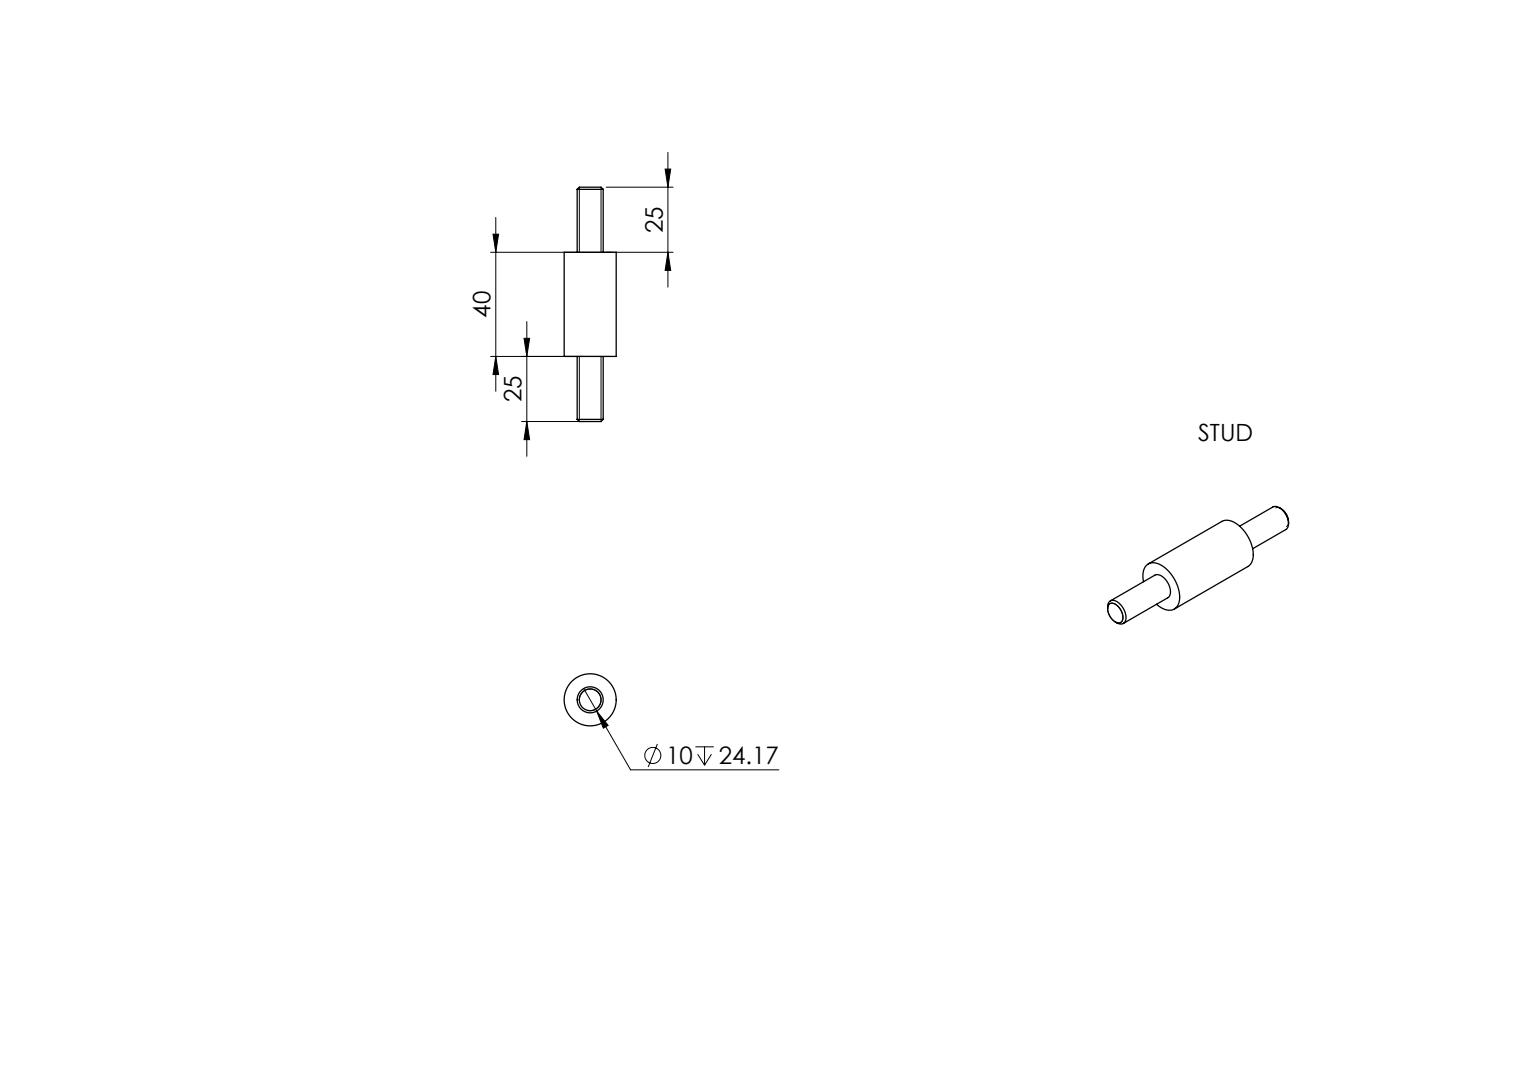
ISO-10303-21;
HEADER;
FILE_DESCRIPTION (('STEP AP214'),
    '1' );
FILE_NAME ('stud.step',
    '2026-10-23T05:12:30',
    ( '' ),
    ( '' ),
    'SwSTEP 2.0',
    'SolidWorks 2026',
    '' );
FILE_SCHEMA (( 'AUTOMOTIVE_DESIGN' ));
ENDSEC;

DATA;
#14=ORIENTED_EDGE ( 'NONE', *, *, #6597, .T. ) ;
#88=ADVANCED_FACE ( 'NONE', ( #7673 ), #6574, .T. ) ;
#119=CIRCLE ( 'NONE', #3022, 10.00000000000000178 ) ;
#120=DIRECTION ( 'NONE',  ( -0.000000000000000000, -0.000000000000000000, 1.000000000000000000 ) ) ;
#168=CIRCLE ( 'NONE', #5710, 4.171999999999995268 ) ;
#219=VERTEX_POINT ( 'NONE', #3065 ) ;
#231=VECTOR ( 'NONE', #6497, 1000.000000000000114 ) ;
#323=EDGE_CURVE ( 'NONE', #1642, #5517, #7754, .T. ) ;
#327=EDGE_CURVE ( 'NONE', #2220, #7617, #7205, .T. ) ;
#347=( LENGTH_UNIT ( ) NAMED_UNIT ( * ) SI_UNIT ( .MILLI., .METRE. ) );
#367=DIRECTION ( 'NONE',  ( -1.000000000000000000, 0.000000000000000000, -0.000000000000000000 ) ) ;
#370=FACE_OUTER_BOUND ( 'NONE', #7061, .T. ) ;
#397=AXIS2_PLACEMENT_3D ( 'NONE', #1905, #4302, #3091 ) ;
#436=DIRECTION ( 'NONE',  ( 0.7071067811865504593, 8.659560562354968603E-17, -0.7071067811865445751 ) ) ;
#446=DIRECTION ( 'NONE',  ( 1.000000000000000000, 0.000000000000000000, 0.000000000000000000 ) ) ;
#447=ORIENTED_EDGE ( 'NONE', *, *, #323, .F. ) ;
#465=ORIENTED_EDGE ( 'NONE', *, *, #7115, .F. ) ;
#478=DIRECTION ( 'NONE',  ( 1.000000000000000000, 0.000000000000000000, -0.000000000000000000 ) ) ;
#535=CIRCLE ( 'NONE', #660, 4.999999999999990230 ) ;
#579=CARTESIAN_POINT ( 'NONE',  ( -68.76644452187068168, 49.96174644486002592, 0.000000000000000000 ) ) ;
#630=( GEOMETRIC_REPRESENTATION_CONTEXT ( 3 ) GLOBAL_UNCERTAINTY_ASSIGNED_CONTEXT ( ( #1956 ) ) GLOBAL_UNIT_ASSIGNED_CONTEXT ( ( #5597, #5554, #3667 ) ) REPRESENTATION_CONTEXT ( 'NONE', 'WORKASPACE' ) );
#641=DIRECTION ( 'NONE',  ( 0.000000000000000000, 0.000000000000000000, 1.000000000000000000 ) ) ;
#660=AXIS2_PLACEMENT_3D ( 'NONE', #1803, #3650, #4750 ) ;
#662=EDGE_CURVE ( 'NONE', #1120, #6644, #7383, .T. ) ;
#676=CONICAL_SURFACE ( 'NONE', #6724, 4.999999999999990230, 0.7853981633974524978 ) ;
#687=DIRECTION ( 'NONE',  ( -0.000000000000000000, -0.000000000000000000, 1.000000000000000000 ) ) ;
#696=CARTESIAN_POINT ( 'NONE',  ( -73.76644452187066747, 49.96174644486002592, 24.17200000000001125 ) ) ;
#697=CARTESIAN_POINT ( 'NONE',  ( -68.76644452187068168, 49.96174644486002592, -40.00000000000000000 ) ) ;
#705=EDGE_CURVE ( 'NONE', #219, #1120, #6679, .T. ) ;
#717=ORIENTED_EDGE ( 'NONE', *, *, #5240, .F. ) ;
#743=VECTOR ( 'NONE', #6568, 1000.000000000000114 ) ;
#771=SHAPE_DEFINITION_REPRESENTATION ( #1259, #2051 ) ;
#773=EDGE_LOOP ( 'NONE', ( #447, #3094 ) ) ;
#801=DIRECTION ( 'NONE',  ( -0.000000000000000000, -0.000000000000000000, -1.000000000000000000 ) ) ;
#805=DIRECTION ( 'NONE',  ( 0.000000000000000000, 0.000000000000000000, 1.000000000000000000 ) ) ;
#838=ORIENTED_EDGE ( 'NONE', *, *, #4223, .T. ) ;
#940=( NAMED_UNIT ( * ) SI_UNIT ( $, .STERADIAN. ) SOLID_ANGLE_UNIT ( ) );
#953=AXIS2_PLACEMENT_3D ( 'NONE', #5493, #7311, #4822 ) ;
#1005=CARTESIAN_POINT ( 'NONE',  ( -63.76644452187068879, 49.96174644486002592, -64.17200000000001125 ) ) ;
#1031=CIRCLE ( 'NONE', #397, 5.000000000000004441 ) ;
#1033=CARTESIAN_POINT ( 'NONE',  ( -68.76644452187068168, 49.96174644486002592, -64.17200000000001125 ) ) ;
#1042=AXIS2_PLACEMENT_3D ( 'NONE', #3660, #3625, #3111 ) ;
#1066=FACE_BOUND ( 'NONE', #2917, .T. ) ;
#1083=ORIENTED_EDGE ( 'NONE', *, *, #6074, .T. ) ;
#1120=VERTEX_POINT ( 'NONE', #1473 ) ;
#1122=ORIENTED_EDGE ( 'NONE', *, *, #7750, .F. ) ;
#1136=DIRECTION ( 'NONE',  ( 1.000000000000000000, 0.000000000000000000, -0.000000000000000000 ) ) ;
#1150=ORIENTED_EDGE ( 'NONE', *, *, #705, .T. ) ;
#1169=CONICAL_SURFACE ( 'NONE', #1042, 4.999999999999990230, 0.7853981633974482790 ) ;
#1183=EDGE_CURVE ( 'NONE', #3506, #5913, #2614, .T. ) ;
#1251=ORIENTED_EDGE ( 'NONE', *, *, #2890, .T. ) ;
#1252=VECTOR ( 'NONE', #3777, 1000.000000000000000 ) ;
#1259=PRODUCT_DEFINITION_SHAPE ( 'NONE', 'NONE',  #6003 ) ;
#1269=CIRCLE ( 'NONE', #1652, 4.171999999999995268 ) ;
#1285=LINE ( 'NONE', #696, #1252 ) ;
#1296=DIRECTION ( 'NONE',  ( -0.000000000000000000, -0.000000000000000000, 1.000000000000000000 ) ) ;
#1301=CARTESIAN_POINT ( 'NONE',  ( 0.000000000000000000, 0.000000000000000000, 0.000000000000000000 ) ) ;
#1309=CARTESIAN_POINT ( 'NONE',  ( -73.76644452187066747, 49.96174644486002592, -40.00000000000000000 ) ) ;
#1337=VERTEX_POINT ( 'NONE', #5175 ) ;
#1338=CARTESIAN_POINT ( 'NONE',  ( -68.76644452187068168, 49.96174644486002592, -40.00000000000000000 ) ) ;
#1369=VECTOR ( 'NONE', #2478, 1000.000000000000000 ) ;
#1381=DIRECTION ( 'NONE',  ( -1.000000000000000000, 0.000000000000000000, 0.000000000000000000 ) ) ;
#1410=ORIENTED_EDGE ( 'NONE', *, *, #6203, .T. ) ;
#1414=( NAMED_UNIT ( * ) PLANE_ANGLE_UNIT ( ) SI_UNIT ( $, .RADIAN. ) );
#1428=VERTEX_POINT ( 'NONE', #4205 ) ;
#1447=ORIENTED_EDGE ( 'NONE', *, *, #4957, .T. ) ;
#1458=FILL_AREA_STYLE_COLOUR ( '', #7110 ) ;
#1473=CARTESIAN_POINT ( 'NONE',  ( -73.76644452187068168, 49.96174644486002592, -40.00000000000000000 ) ) ;
#1510=CARTESIAN_POINT ( 'NONE',  ( -68.76644452187068168, 49.96174644486002592, 25.00000000000000000 ) ) ;
#1538=DIRECTION ( 'NONE',  ( -0.000000000000000000, -0.000000000000000000, -1.000000000000000000 ) ) ;
#1548=ORIENTED_EDGE ( 'NONE', *, *, #7688, .F. ) ;
#1640=ORIENTED_EDGE ( 'NONE', *, *, #6203, .F. ) ;
#1642=VERTEX_POINT ( 'NONE', #3296 ) ;
#1652=AXIS2_PLACEMENT_3D ( 'NONE', #3931, #2716, #7556 ) ;
#1678=DIRECTION ( 'NONE',  ( 0.000000000000000000, 0.000000000000000000, 1.000000000000000000 ) ) ;
#1688=EDGE_CURVE ( 'NONE', #3738, #1337, #2044, .T. ) ;
#1699=CARTESIAN_POINT ( 'NONE',  ( -68.76644452187068168, 49.96174644486002592, -40.00000000000000000 ) ) ;
#1746=FACE_BOUND ( 'NONE', #3075, .T. ) ;
#1756=CARTESIAN_POINT ( 'NONE',  ( -63.76644452187067458, 49.96174644486002592, -40.00000000000000000 ) ) ;
#1768=ORIENTED_EDGE ( 'NONE', *, *, #4275, .F. ) ;
#1776=FACE_OUTER_BOUND ( 'NONE', #6687, .T. ) ;
#1785=CARTESIAN_POINT ( 'NONE',  ( -68.76644452187068168, 49.96174644486002592, -40.00000000000000000 ) ) ;
#1787=DIRECTION ( 'NONE',  ( -0.000000000000000000, -0.000000000000000000, -1.000000000000000000 ) ) ;
#1792=PLANE ( 'NONE',  #3043 ) ;
#1803=CARTESIAN_POINT ( 'NONE',  ( -68.76644452187068168, 49.96174644486002592, 24.17200000000001125 ) ) ;
#1808=CARTESIAN_POINT ( 'NONE',  ( -63.76644452187068879, 49.96174644486002592, 0.000000000000000000 ) ) ;
#1851=UNCERTAINTY_MEASURE_WITH_UNIT (LENGTH_MEASURE( 1.000000000000000082E-05 ), #347, 'distance_accuracy_value', 'NONE');
#1905=CARTESIAN_POINT ( 'NONE',  ( -68.76644452187068168, 49.96174644486002592, 0.000000000000000000 ) ) ;
#1906=EDGE_LOOP ( 'NONE', ( #7125, #6227, #1640, #4041 ) ) ;
#1944=CARTESIAN_POINT ( 'NONE',  ( -68.76644452187068168, 49.96174644486002592, 24.17200000000001125 ) ) ;
#1956=UNCERTAINTY_MEASURE_WITH_UNIT (LENGTH_MEASURE( 1.000000000000000082E-05 ), #5597, 'distance_accuracy_value', 'NONE');
#1970=DIRECTION ( 'NONE',  ( 1.000000000000000000, 0.000000000000000000, 0.000000000000000000 ) ) ;
#1998=EDGE_LOOP ( 'NONE', ( #2681, #1447, #3493, #1768 ) ) ;
#2000=VECTOR ( 'NONE', #436, 1000.000000000000000 ) ;
#2026=FILL_AREA_STYLE ('',( #1458 ) ) ;
#2044=LINE ( 'NONE', #4437, #2119 ) ;
#2051=SHAPE_REPRESENTATION ( 'stud', ( #7485 ), #2832 ) ;
#2072=AXIS2_PLACEMENT_3D ( 'NONE', #1699, #3429, #7580 ) ;
#2076=EDGE_LOOP ( 'NONE', ( #2825, #2305 ) ) ;
#2099=PRODUCT ( 'stud', 'stud', '', ( #6182 ) ) ;
#2119=VECTOR ( 'NONE', #805, 1000.000000000000000 ) ;
#2195=CARTESIAN_POINT ( 'NONE',  ( -63.76644452187067458, 49.96174644486002592, 0.000000000000000000 ) ) ;
#2203=EDGE_LOOP ( 'NONE', ( #6601, #838, #1251, #717 ) ) ;
#2205=DIRECTION ( 'NONE',  ( -0.000000000000000000, -0.000000000000000000, -1.000000000000000000 ) ) ;
#2206=AXIS2_PLACEMENT_3D ( 'NONE', #4634, #1678, #7583 ) ;
#2220=VERTEX_POINT ( 'NONE', #4542 ) ;
#2223=( NAMED_UNIT ( * ) SI_UNIT ( $, .STERADIAN. ) SOLID_ANGLE_UNIT ( ) );
#2232=CARTESIAN_POINT ( 'NONE',  ( -63.76644452187068879, 49.96174644486002592, 24.17200000000001125 ) ) ;
#2240=CARTESIAN_POINT ( 'NONE',  ( -64.59444452187068464, 49.96174644486002592, -65.00000000000000000 ) ) ;
#2279=EDGE_CURVE ( 'NONE', #5913, #2220, #6518, .T. ) ;
#2305=ORIENTED_EDGE ( 'NONE', *, *, #4893, .T. ) ;
#2308=CARTESIAN_POINT ( 'NONE',  ( -68.76644452187068168, 49.96174644486002592, 0.000000000000000000 ) ) ;
#2321=CARTESIAN_POINT ( 'NONE',  ( -68.76644452187068168, 49.96174644486002592, -65.00000000000000000 ) ) ;
#2360=CARTESIAN_POINT ( 'NONE',  ( -68.76644452187068168, 49.96174644486002592, 0.000000000000000000 ) ) ;
#2406=DIRECTION ( 'NONE',  ( 1.000000000000000000, 0.000000000000000000, 0.000000000000000000 ) ) ;
#2431=ORIENTED_EDGE ( 'NONE', *, *, #4223, .F. ) ;
#2446=APPLICATION_CONTEXT ( 'automotive_design' ) ;
#2449=CIRCLE ( 'NONE', #6594, 10.00000000000000178 ) ;
#2473=VECTOR ( 'NONE', #687, 1000.000000000000000 ) ;
#2478=DIRECTION ( 'NONE',  ( 0.000000000000000000, 0.000000000000000000, 1.000000000000000000 ) ) ;
#2520=CIRCLE ( 'NONE', #3394, 10.00000000000000178 ) ;
#2541=DIRECTION ( 'NONE',  ( -0.000000000000000000, -0.000000000000000000, 1.000000000000000000 ) ) ;
#2542=FACE_OUTER_BOUND ( 'NONE', #1906, .T. ) ;
#2554=ADVANCED_FACE ( 'NONE', ( #2542 ), #3635, .T. ) ;
#2573=DIRECTION ( 'NONE',  ( 1.000000000000000000, 0.000000000000000000, 0.000000000000000000 ) ) ;
#2614=CIRCLE ( 'NONE', #2730, 4.171999999999995268 ) ;
#2681=ORIENTED_EDGE ( 'NONE', *, *, #323, .T. ) ;
#2692=AXIS2_PLACEMENT_3D ( 'NONE', #697, #4954, #1970 ) ;
#2704=CARTESIAN_POINT ( 'NONE',  ( -68.76644452187068168, 49.96174644486002592, 0.000000000000000000 ) ) ;
#2716=DIRECTION ( 'NONE',  ( -0.000000000000000000, -0.000000000000000000, -1.000000000000000000 ) ) ;
#2723=CARTESIAN_POINT ( 'NONE',  ( -63.76644452187068879, 49.96174644486002592, -64.17200000000001125 ) ) ;
#2730=AXIS2_PLACEMENT_3D ( 'NONE', #1510, #801, #5025 ) ;
#2747=ORIENTED_EDGE ( 'NONE', *, *, #6074, .F. ) ;
#2759=CARTESIAN_POINT ( 'NONE',  ( -72.93844452187067873, 49.96174644486002592, -65.00000000000000000 ) ) ;
#2796=LINE ( 'NONE', #1005, #231 ) ;
#2797=FACE_OUTER_BOUND ( 'NONE', #3560, .T. ) ;
#2799=DIRECTION ( 'NONE',  ( 1.000000000000000000, 0.000000000000000000, 0.000000000000000000 ) ) ;
#2819=DIRECTION ( 'NONE',  ( -0.000000000000000000, -0.000000000000000000, -1.000000000000000000 ) ) ;
#2825=ORIENTED_EDGE ( 'NONE', *, *, #7176, .T. ) ;
#2832=( GEOMETRIC_REPRESENTATION_CONTEXT ( 3 ) GLOBAL_UNCERTAINTY_ASSIGNED_CONTEXT ( ( #1851 ) ) GLOBAL_UNIT_ASSIGNED_CONTEXT ( ( #347, #1414, #940 ) ) REPRESENTATION_CONTEXT ( 'NONE', 'WORKASPACE' ) );
#2869=DIRECTION ( 'NONE',  ( -1.000000000000000000, 0.000000000000000000, 0.000000000000000000 ) ) ;
#2890=EDGE_CURVE ( 'NONE', #3506, #3664, #1285, .T. ) ;
#2892=CARTESIAN_POINT ( 'NONE',  ( -72.93844452187067873, 49.96174644486002592, 25.00000000000000000 ) ) ;
#2902=DIRECTION ( 'NONE',  ( 0.000000000000000000, 0.000000000000000000, -1.000000000000000000 ) ) ;
#2906=EDGE_LOOP ( 'NONE', ( #1410, #6235, #1548, #5258 ) ) ;
#2917=EDGE_LOOP ( 'NONE', ( #6895, #14 ) ) ;
#2922=SHAPE_REPRESENTATION_RELATIONSHIP ( 'NONE' , 'NONE' ,  #2051, #5395 ) ;
#2933=FACE_OUTER_BOUND ( 'NONE', #3193, .T. ) ;
#2935=ORIENTED_EDGE ( 'NONE', *, *, #5238, .T. ) ;
#2958=ORIENTED_EDGE ( 'NONE', *, *, #4275, .T. ) ;
#3004=CARTESIAN_POINT ( 'NONE',  ( -68.76644452187068168, 49.96174644486002592, -40.00000000000000000 ) ) ;
#3022=AXIS2_PLACEMENT_3D ( 'NONE', #3004, #7723, #4095 ) ;
#3043=AXIS2_PLACEMENT_3D ( 'NONE', #2308, #7729, #478 ) ;
#3045=FACE_OUTER_BOUND ( 'NONE', #7561, .T. ) ;
#3065=CARTESIAN_POINT ( 'NONE',  ( -73.76644452187066747, 49.96174644486002592, -64.17200000000001125 ) ) ;
#3075=EDGE_LOOP ( 'NONE', ( #6128, #4726 ) ) ;
#3081=ADVANCED_FACE ( 'NONE', ( #1746, #3045 ), #7179, .F. ) ;
#3089=AXIS2_PLACEMENT_3D ( 'NONE', #1033, #2541, #7117 ) ;
#3091=DIRECTION ( 'NONE',  ( -1.000000000000000000, 0.000000000000000000, 0.000000000000000000 ) ) ;
#3093=EDGE_CURVE ( 'NONE', #3738, #4221, #119, .T. ) ;
#3094=ORIENTED_EDGE ( 'NONE', *, *, #5388, .F. ) ;
#3111=DIRECTION ( 'NONE',  ( 1.000000000000000000, 0.000000000000000000, 0.000000000000000000 ) ) ;
#3183=MANIFOLD_SOLID_BREP ( 'Mirror1', #5858 ) ;
#3193=EDGE_LOOP ( 'NONE', ( #6194, #2431 ) ) ;
#3280=FACE_OUTER_BOUND ( 'NONE', #2203, .T. ) ;
#3296=CARTESIAN_POINT ( 'NONE',  ( -64.59444452187068464, 49.96174644486002592, -65.00000000000000000 ) ) ;
#3360=ADVANCED_FACE ( 'NONE', ( #2797 ), #4604, .T. ) ;
#3394=AXIS2_PLACEMENT_3D ( 'NONE', #2360, #5978, #4862 ) ;
#3402=STYLED_ITEM('',(#7837),#3183);
#3420=DIRECTION ( 'NONE',  ( 1.000000000000000000, 0.000000000000000000, 0.000000000000000000 ) ) ;
#3429=DIRECTION ( 'NONE',  ( 0.000000000000000000, 0.000000000000000000, 1.000000000000000000 ) ) ;
#3441=ORIENTED_EDGE ( 'NONE', *, *, #705, .F. ) ;
#3450=CONICAL_SURFACE ( 'NONE', #4834, 4.999999999999990230, 0.7853981633974482790 ) ;
#3469=VERTEX_POINT ( 'NONE', #4659 ) ;
#3475=ORIENTED_EDGE ( 'NONE', *, *, #7750, .T. ) ;
#3478=FACE_OUTER_BOUND ( 'NONE', #2076, .T. ) ;
#3493=ORIENTED_EDGE ( 'NONE', *, *, #7127, .F. ) ;
#3504=ADVANCED_FACE ( 'NONE', ( #1066, #3478 ), #1792, .T. ) ;
#3506=VERTEX_POINT ( 'NONE', #2892 ) ;
#3514=ADVANCED_FACE ( 'NONE', ( #4622 ), #4852, .T. ) ;
#3548=( LENGTH_UNIT ( ) NAMED_UNIT ( * ) SI_UNIT ( .MILLI., .METRE. ) );
#3550=CARTESIAN_POINT ( 'NONE',  ( -68.76644452187068168, 49.96174644486002592, 24.17200000000001125 ) ) ;
#3560=EDGE_LOOP ( 'NONE', ( #5361, #7522, #5267, #7410 ) ) ;
#3564=ORIENTED_EDGE ( 'NONE', *, *, #4947, .F. ) ;
#3572=LINE ( 'NONE', #6058, #2473 ) ;
#3625=DIRECTION ( 'NONE',  ( -0.000000000000000000, -0.000000000000000000, 1.000000000000000000 ) ) ;
#3635=CONICAL_SURFACE ( 'NONE', #7154, 4.999999999999990230, 0.7853981633974524978 ) ;
#3641=AXIS2_PLACEMENT_3D ( 'NONE', #2240, #2902, #367 ) ;
#3650=DIRECTION ( 'NONE',  ( -0.000000000000000000, -0.000000000000000000, -1.000000000000000000 ) ) ;
#3660=CARTESIAN_POINT ( 'NONE',  ( -68.76644452187068168, 49.96174644486002592, -64.17200000000001125 ) ) ;
#3664=VERTEX_POINT ( 'NONE', #3979 ) ;
#3667=( NAMED_UNIT ( * ) SI_UNIT ( $, .STERADIAN. ) SOLID_ANGLE_UNIT ( ) );
#3671=VERTEX_POINT ( 'NONE', #2723 ) ;
#3696=AXIS2_PLACEMENT_3D ( 'NONE', #6524, #7197, #5976 ) ;
#3722=DIRECTION ( 'NONE',  ( -0.000000000000000000, -0.000000000000000000, 1.000000000000000000 ) ) ;
#3738=VERTEX_POINT ( 'NONE', #7452 ) ;
#3758=DIRECTION ( 'NONE',  ( 0.000000000000000000, 0.000000000000000000, 1.000000000000000000 ) ) ;
#3777=DIRECTION ( 'NONE',  ( -0.7071067811865504593, 0.000000000000000000, -0.7071067811865445751 ) ) ;
#3828=AXIS2_PLACEMENT_3D ( 'NONE', #3550, #7724, #5836 ) ;
#3830=SURFACE_STYLE_FILL_AREA ( #2026 ) ;
#3899=DIRECTION ( 'NONE',  ( 0.000000000000000000, 0.000000000000000000, 1.000000000000000000 ) ) ;
#3923=CARTESIAN_POINT ( 'NONE',  ( -64.59444452187068464, 49.96174644486002592, 25.00000000000000000 ) ) ;
#3931=CARTESIAN_POINT ( 'NONE',  ( -68.76644452187068168, 49.96174644486002592, 25.00000000000000000 ) ) ;
#3949=ORIENTED_EDGE ( 'NONE', *, *, #5238, .F. ) ;
#3979=CARTESIAN_POINT ( 'NONE',  ( -73.76644452187066747, 49.96174644486002592, 24.17200000000001125 ) ) ;
#4000=DIRECTION ( 'NONE',  ( -0.000000000000000000, -0.000000000000000000, 1.000000000000000000 ) ) ;
#4017=SURFACE_STYLE_USAGE ( .BOTH. , #6237 ) ;
#4041=ORIENTED_EDGE ( 'NONE', *, *, #2890, .F. ) ;
#4053=( NAMED_UNIT ( * ) PLANE_ANGLE_UNIT ( ) SI_UNIT ( $, .RADIAN. ) );
#4095=DIRECTION ( 'NONE',  ( 1.000000000000000000, 0.000000000000000000, 0.000000000000000000 ) ) ;
#4115=CYLINDRICAL_SURFACE ( 'NONE', #2206, 10.00000000000000178 ) ;
#4167=DIRECTION ( 'NONE',  ( -0.000000000000000000, -0.000000000000000000, 1.000000000000000000 ) ) ;
#4205=CARTESIAN_POINT ( 'NONE',  ( -73.76644452187068168, 49.96174644486002592, 0.000000000000000000 ) ) ;
#4221=VERTEX_POINT ( 'NONE', #5634 ) ;
#4223=EDGE_CURVE ( 'NONE', #5913, #3506, #1269, .T. ) ;
#4233=LINE ( 'NONE', #7156, #1369 ) ;
#4239=DIRECTION ( 'NONE',  ( -0.000000000000000000, -0.000000000000000000, 1.000000000000000000 ) ) ;
#4275=EDGE_CURVE ( 'NONE', #1642, #3671, #2796, .T. ) ;
#4287=AXIS2_PLACEMENT_3D ( 'NONE', #1338, #120, #5448 ) ;
#4302=DIRECTION ( 'NONE',  ( -0.000000000000000000, -0.000000000000000000, -1.000000000000000000 ) ) ;
#4335=ORIENTED_EDGE ( 'NONE', *, *, #4957, .F. ) ;
#4437=CARTESIAN_POINT ( 'NONE',  ( -78.76644452187068168, 49.96174644486002592, -40.00000000000000000 ) ) ;
#4463=CIRCLE ( 'NONE', #3089, 4.999999999999990230 ) ;
#4470=AXIS2_PLACEMENT_3D ( 'NONE', #5264, #4000, #446 ) ;
#4537=ORIENTED_EDGE ( 'NONE', *, *, #5388, .T. ) ;
#4542=CARTESIAN_POINT ( 'NONE',  ( -63.76644452187068879, 49.96174644486002592, 24.17200000000001125 ) ) ;
#4604=CYLINDRICAL_SURFACE ( 'NONE', #6809, 10.00000000000000178 ) ;
#4622=FACE_OUTER_BOUND ( 'NONE', #5873, .T. ) ;
#4634=CARTESIAN_POINT ( 'NONE',  ( -68.76644452187068168, 49.96174644486002592, -40.00000000000000000 ) ) ;
#4659=CARTESIAN_POINT ( 'NONE',  ( -58.76644452187068168, 49.96174644486002592, 0.000000000000000000 ) ) ;
#4679=CARTESIAN_POINT ( 'NONE',  ( -68.76644452187068168, 49.96174644486002592, -64.17200000000001125 ) ) ;
#4710=PRODUCT_DEFINITION_CONTEXT ( 'detailed design', #7516, 'design' ) ;
#4726=ORIENTED_EDGE ( 'NONE', *, *, #662, .T. ) ;
#4746=LINE ( 'NONE', #6015, #743 ) ;
#4750=DIRECTION ( 'NONE',  ( -1.000000000000000000, 0.000000000000000000, 0.000000000000000000 ) ) ;
#4794=ADVANCED_FACE ( 'NONE', ( #7581 ), #6960, .T. ) ;
#4822=DIRECTION ( 'NONE',  ( 1.000000000000000000, 0.000000000000000000, 0.000000000000000000 ) ) ;
#4834=AXIS2_PLACEMENT_3D ( 'NONE', #4679, #4167, #2799 ) ;
#4852=CYLINDRICAL_SURFACE ( 'NONE', #4287, 4.999999999999990230 ) ;
#4862=DIRECTION ( 'NONE',  ( 1.000000000000000000, 0.000000000000000000, 0.000000000000000000 ) ) ;
#4869=VECTOR ( 'NONE', #3722, 1000.000000000000000 ) ;
#4893=EDGE_CURVE ( 'NONE', #1337, #3469, #2520, .T. ) ;
#4947=EDGE_CURVE ( 'NONE', #4221, #3469, #4233, .T. ) ;
#4954=DIRECTION ( 'NONE',  ( -0.000000000000000000, -0.000000000000000000, 1.000000000000000000 ) ) ;
#4957=EDGE_CURVE ( 'NONE', #5517, #219, #4746, .T. ) ;
#4959=CIRCLE ( 'NONE', #2072, 10.00000000000000178 ) ;
#5025=DIRECTION ( 'NONE',  ( -1.000000000000000000, 0.000000000000000000, 0.000000000000000000 ) ) ;
#5027=AXIS2_PLACEMENT_3D ( 'NONE', #1785, #5877, #1136 ) ;
#5068=AXIS2_PLACEMENT_3D ( 'NONE', #5928, #641, #7267 ) ;
#5137=ADVANCED_FACE ( 'NONE', ( #3280 ), #676, .T. ) ;
#5175=CARTESIAN_POINT ( 'NONE',  ( -78.76644452187068168, 49.96174644486002592, 0.000000000000000000 ) ) ;
#5188=EDGE_LOOP ( 'NONE', ( #3441, #3475, #1083, #6863 ) ) ;
#5238=EDGE_CURVE ( 'NONE', #4221, #3738, #4959, .T. ) ;
#5240=EDGE_CURVE ( 'NONE', #2220, #3664, #6469, .T. ) ;
#5244=PRESENTATION_STYLE_ASSIGNMENT (( #4017 ) ) ;
#5258=ORIENTED_EDGE ( 'NONE', *, *, #5282, .F. ) ;
#5264=CARTESIAN_POINT ( 'NONE',  ( -68.76644452187068168, 49.96174644486002592, -40.00000000000000000 ) ) ;
#5267=ORIENTED_EDGE ( 'NONE', *, *, #4947, .T. ) ;
#5282=EDGE_CURVE ( 'NONE', #3664, #1428, #7181, .T. ) ;
#5286=MECHANICAL_DESIGN_GEOMETRIC_PRESENTATION_REPRESENTATION('',(#3402),#630);
#5339=ORIENTED_EDGE ( 'NONE', *, *, #5240, .T. ) ;
#5361=ORIENTED_EDGE ( 'NONE', *, *, #1688, .F. ) ;
#5388=EDGE_CURVE ( 'NONE', #5517, #1642, #168, .T. ) ;
#5395=ADVANCED_BREP_SHAPE_REPRESENTATION ( '', ( #3183, #7485 ), #2832 ) ;
#5448=DIRECTION ( 'NONE',  ( 1.000000000000000000, 0.000000000000000000, 0.000000000000000000 ) ) ;
#5493=CARTESIAN_POINT ( 'NONE',  ( -68.76644452187068168, 49.96174644486002592, -40.00000000000000000 ) ) ;
#5517=VERTEX_POINT ( 'NONE', #2759 ) ;
#5554=( NAMED_UNIT ( * ) PLANE_ANGLE_UNIT ( ) SI_UNIT ( $, .RADIAN. ) );
#5560=ORIENTED_EDGE ( 'NONE', *, *, #7176, .F. ) ;
#5579=ADVANCED_FACE ( 'NONE', ( #7446 ), #6862, .T. ) ;
#5597=( LENGTH_UNIT ( ) NAMED_UNIT ( * ) SI_UNIT ( .MILLI., .METRE. ) );
#5618=AXIS2_PLACEMENT_3D ( 'NONE', #2321, #4239, #2406 ) ;
#5634=CARTESIAN_POINT ( 'NONE',  ( -58.76644452187068168, 49.96174644486002592, -40.00000000000000000 ) ) ;
#5679=DIRECTION ( 'NONE',  ( -1.000000000000000000, 0.000000000000000000, 0.000000000000000000 ) ) ;
#5710=AXIS2_PLACEMENT_3D ( 'NONE', #6040, #1296, #2573 ) ;
#5712=ADVANCED_FACE ( 'NONE', ( #1776 ), #3450, .T. ) ;
#5718=CIRCLE ( 'NONE', #7731, 5.000000000000004441 ) ;
#5733=AXIS2_PLACEMENT_3D ( 'NONE', #579, #2205, #2869 ) ;
#5757=CARTESIAN_POINT ( 'NONE',  ( -68.76644452187068168, 49.96174644486002592, 24.17200000000001125 ) ) ;
#5785=DIRECTION ( 'NONE',  ( 1.000000000000000000, 0.000000000000000000, 0.000000000000000000 ) ) ;
#5834=CIRCLE ( 'NONE', #3696, 4.999999999999990230 ) ;
#5836=DIRECTION ( 'NONE',  ( -1.000000000000000000, 0.000000000000000000, 0.000000000000000000 ) ) ;
#5842=AXIS2_PLACEMENT_3D ( 'NONE', #6901, #6311, #6384 ) ;
#5849=STYLED_ITEM ( 'NONE', ( #5244 ), #5395 ) ;
#5858=CLOSED_SHELL ( 'NONE', ( #3514, #7017, #5579, #2554, #5959, #3360, #3081, #3504, #6705, #5137, #88, #4794, #5712, #6034 ) ) ;
#5859=ORIENTED_EDGE ( 'NONE', *, *, #3093, .F. ) ;
#5873=EDGE_LOOP ( 'NONE', ( #7708, #1150, #465, #2747 ) ) ;
#5877=DIRECTION ( 'NONE',  ( 0.000000000000000000, 0.000000000000000000, 1.000000000000000000 ) ) ;
#5913=VERTEX_POINT ( 'NONE', #3923 ) ;
#5928=CARTESIAN_POINT ( 'NONE',  ( -64.59444452187068464, 49.96174644486002592, 25.00000000000000000 ) ) ;
#5934=CARTESIAN_POINT ( 'NONE',  ( -68.76644452187068168, 49.96174644486002592, 0.000000000000000000 ) ) ;
#5959=ADVANCED_FACE ( 'NONE', ( #370 ), #4115, .T. ) ;
#5967=DIRECTION ( 'NONE',  ( -0.000000000000000000, -0.000000000000000000, -1.000000000000000000 ) ) ;
#5976=DIRECTION ( 'NONE',  ( 1.000000000000000000, 0.000000000000000000, 0.000000000000000000 ) ) ;
#5977=DIRECTION ( 'NONE',  ( 1.000000000000000000, 0.000000000000000000, 0.000000000000000000 ) ) ;
#5978=DIRECTION ( 'NONE',  ( 0.000000000000000000, 0.000000000000000000, 1.000000000000000000 ) ) ;
#5999=CARTESIAN_POINT ( 'NONE',  ( -73.76644452187066747, 49.96174644486002592, 0.000000000000000000 ) ) ;
#6003=PRODUCT_DEFINITION ( 'UNKNOWN', '', #6841, #4710 ) ;
#6015=CARTESIAN_POINT ( 'NONE',  ( -73.76644452187066747, 49.96174644486002592, -64.17200000000001125 ) ) ;
#6034=ADVANCED_FACE ( 'NONE', ( #7122 ), #6529, .T. ) ;
#6040=CARTESIAN_POINT ( 'NONE',  ( -68.76644452187068168, 49.96174644486002592, -65.00000000000000000 ) ) ;
#6047=PLANE ( 'NONE',  #5068 ) ;
#6058=CARTESIAN_POINT ( 'NONE',  ( -63.76644452187068879, 49.96174644486002592, -40.00000000000000000 ) ) ;
#6074=EDGE_CURVE ( 'NONE', #3671, #6644, #3572, .T. ) ;
#6118=ORIENTED_EDGE ( 'NONE', *, *, #1688, .T. ) ;
#6128=ORIENTED_EDGE ( 'NONE', *, *, #7115, .T. ) ;
#6182=PRODUCT_CONTEXT ( 'NONE', #2446, 'mechanical' ) ;
#6194=ORIENTED_EDGE ( 'NONE', *, *, #1183, .F. ) ;
#6203=EDGE_CURVE ( 'NONE', #3664, #2220, #535, .T. ) ;
#6227=ORIENTED_EDGE ( 'NONE', *, *, #2279, .T. ) ;
#6235=ORIENTED_EDGE ( 'NONE', *, *, #327, .T. ) ;
#6237=SURFACE_SIDE_STYLE ('',( #3830 ) ) ;
#6311=DIRECTION ( 'NONE',  ( -0.000000000000000000, -0.000000000000000000, -1.000000000000000000 ) ) ;
#6314=ORIENTED_EDGE ( 'NONE', *, *, #6597, .F. ) ;
#6331=DIRECTION ( 'NONE',  ( -1.000000000000000000, 0.000000000000000000, 0.000000000000000000 ) ) ;
#6343=CARTESIAN_POINT ( 'NONE',  ( -68.76644452187068168, 49.96174644486002592, -40.00000000000000000 ) ) ;
#6360=( GEOMETRIC_REPRESENTATION_CONTEXT ( 3 ) GLOBAL_UNCERTAINTY_ASSIGNED_CONTEXT ( ( #7288 ) ) GLOBAL_UNIT_ASSIGNED_CONTEXT ( ( #3548, #4053, #2223 ) ) REPRESENTATION_CONTEXT ( 'NONE', 'WORKASPACE' ) );
#6384=DIRECTION ( 'NONE',  ( -1.000000000000000000, 0.000000000000000000, 0.000000000000000000 ) ) ;
#6469=CIRCLE ( 'NONE', #3828, 4.999999999999990230 ) ;
#6497=DIRECTION ( 'NONE',  ( 0.7071067811865474617, 0.000000000000000000, 0.7071067811865474617 ) ) ;
#6512=FACE_OUTER_BOUND ( 'NONE', #1998, .T. ) ;
#6518=LINE ( 'NONE', #2232, #2000 ) ;
#6524=CARTESIAN_POINT ( 'NONE',  ( -68.76644452187068168, 49.96174644486002592, -64.17200000000001125 ) ) ;
#6529=CYLINDRICAL_SURFACE ( 'NONE', #4470, 4.999999999999990230 ) ;
#6568=DIRECTION ( 'NONE',  ( -0.7071067811865474617, 8.659560562354932858E-17, 0.7071067811865474617 ) ) ;
#6574=CYLINDRICAL_SURFACE ( 'NONE', #5733, 4.999999999999990230 ) ;
#6594=AXIS2_PLACEMENT_3D ( 'NONE', #5934, #6969, #5785 ) ;
#6597=EDGE_CURVE ( 'NONE', #7617, #1428, #1031, .T. ) ;
#6601=ORIENTED_EDGE ( 'NONE', *, *, #2279, .F. ) ;
#6644=VERTEX_POINT ( 'NONE', #1756 ) ;
#6653=DIRECTION ( 'NONE',  ( -0.000000000000000000, -0.000000000000000000, -1.000000000000000000 ) ) ;
#6675=ORIENTED_EDGE ( 'NONE', *, *, #327, .F. ) ;
#6679=LINE ( 'NONE', #1309, #4869 ) ;
#6687=EDGE_LOOP ( 'NONE', ( #4335, #4537, #2958, #1122 ) ) ;
#6705=ADVANCED_FACE ( 'NONE', ( #2933 ), #6047, .T. ) ;
#6724=AXIS2_PLACEMENT_3D ( 'NONE', #5757, #1538, #5679 ) ;
#6758=VECTOR ( 'NONE', #6653, 1000.000000000000000 ) ;
#6809=AXIS2_PLACEMENT_3D ( 'NONE', #6343, #3899, #3420 ) ;
#6841=PRODUCT_DEFINITION_FORMATION_WITH_SPECIFIED_SOURCE ( 'ANY', '', #2099, .NOT_KNOWN. ) ;
#6854=VECTOR ( 'NONE', #1787, 1000.000000000000000 ) ;
#6862=CYLINDRICAL_SURFACE ( 'NONE', #5842, 4.999999999999990230 ) ;
#6863=ORIENTED_EDGE ( 'NONE', *, *, #662, .F. ) ;
#6895=ORIENTED_EDGE ( 'NONE', *, *, #7688, .T. ) ;
#6901=CARTESIAN_POINT ( 'NONE',  ( -68.76644452187068168, 49.96174644486002592, 0.000000000000000000 ) ) ;
#6960=PLANE ( 'NONE',  #3641 ) ;
#6969=DIRECTION ( 'NONE',  ( 0.000000000000000000, 0.000000000000000000, 1.000000000000000000 ) ) ;
#7017=ADVANCED_FACE ( 'NONE', ( #6512 ), #1169, .T. ) ;
#7061=EDGE_LOOP ( 'NONE', ( #2935, #6118, #5560, #3564 ) ) ;
#7110=COLOUR_RGB ( '',0.8941176470588234615, 0.8941176470588234615, 0.8941176470588234615 ) ;
#7115=EDGE_CURVE ( 'NONE', #6644, #1120, #7587, .T. ) ;
#7117=DIRECTION ( 'NONE',  ( 1.000000000000000000, 0.000000000000000000, 0.000000000000000000 ) ) ;
#7122=FACE_OUTER_BOUND ( 'NONE', #5188, .T. ) ;
#7125=ORIENTED_EDGE ( 'NONE', *, *, #1183, .T. ) ;
#7127=EDGE_CURVE ( 'NONE', #3671, #219, #5834, .T. ) ;
#7154=AXIS2_PLACEMENT_3D ( 'NONE', #1944, #5967, #1381 ) ;
#7156=CARTESIAN_POINT ( 'NONE',  ( -58.76644452187068168, 49.96174644486002592, -40.00000000000000000 ) ) ;
#7176=EDGE_CURVE ( 'NONE', #3469, #1337, #2449, .T. ) ;
#7179=PLANE ( 'NONE',  #5027 ) ;
#7181=LINE ( 'NONE', #5999, #6854 ) ;
#7197=DIRECTION ( 'NONE',  ( -0.000000000000000000, -0.000000000000000000, 1.000000000000000000 ) ) ;
#7205=LINE ( 'NONE', #1808, #6758 ) ;
#7243=MECHANICAL_DESIGN_GEOMETRIC_PRESENTATION_REPRESENTATION('',(#5849),#6360);
#7267=DIRECTION ( 'NONE',  ( 1.000000000000000000, 0.000000000000000000, -0.000000000000000000 ) ) ;
#7288=UNCERTAINTY_MEASURE_WITH_UNIT (LENGTH_MEASURE( 1.000000000000000082E-05 ), #3548, 'distance_accuracy_value', 'NONE');
#7311=DIRECTION ( 'NONE',  ( -0.000000000000000000, -0.000000000000000000, 1.000000000000000000 ) ) ;
#7382=EDGE_LOOP ( 'NONE', ( #6675, #5339, #7668, #6314 ) ) ;
#7383=CIRCLE ( 'NONE', #953, 5.000000000000004441 ) ;
#7410=ORIENTED_EDGE ( 'NONE', *, *, #4893, .F. ) ;
#7446=FACE_OUTER_BOUND ( 'NONE', #2906, .T. ) ;
#7452=CARTESIAN_POINT ( 'NONE',  ( -78.76644452187068168, 49.96174644486002592, -40.00000000000000000 ) ) ;
#7485=AXIS2_PLACEMENT_3D ( 'NONE', #1301, #3758, #5977 ) ;
#7516=APPLICATION_CONTEXT ( 'automotive_design' ) ;
#7522=ORIENTED_EDGE ( 'NONE', *, *, #3093, .T. ) ;
#7556=DIRECTION ( 'NONE',  ( -1.000000000000000000, 0.000000000000000000, 0.000000000000000000 ) ) ;
#7561=EDGE_LOOP ( 'NONE', ( #3949, #5859 ) ) ;
#7580=DIRECTION ( 'NONE',  ( 1.000000000000000000, 0.000000000000000000, 0.000000000000000000 ) ) ;
#7581=FACE_OUTER_BOUND ( 'NONE', #773, .T. ) ;
#7583=DIRECTION ( 'NONE',  ( 1.000000000000000000, 0.000000000000000000, 0.000000000000000000 ) ) ;
#7587=CIRCLE ( 'NONE', #2692, 5.000000000000004441 ) ;
#7617=VERTEX_POINT ( 'NONE', #2195 ) ;
#7668=ORIENTED_EDGE ( 'NONE', *, *, #5282, .T. ) ;
#7673=FACE_OUTER_BOUND ( 'NONE', #7382, .T. ) ;
#7688=EDGE_CURVE ( 'NONE', #1428, #7617, #5718, .T. ) ;
#7708=ORIENTED_EDGE ( 'NONE', *, *, #7127, .T. ) ;
#7723=DIRECTION ( 'NONE',  ( 0.000000000000000000, 0.000000000000000000, 1.000000000000000000 ) ) ;
#7724=DIRECTION ( 'NONE',  ( -0.000000000000000000, -0.000000000000000000, -1.000000000000000000 ) ) ;
#7729=DIRECTION ( 'NONE',  ( 0.000000000000000000, 0.000000000000000000, 1.000000000000000000 ) ) ;
#7731=AXIS2_PLACEMENT_3D ( 'NONE', #2704, #2819, #6331 ) ;
#7750=EDGE_CURVE ( 'NONE', #219, #3671, #4463, .T. ) ;
#7754=CIRCLE ( 'NONE', #5618, 4.171999999999995268 ) ;
#7831=COLOUR_RGB('Black',0.12,0.14,0.17);
#7832=FILL_AREA_STYLE_COLOUR('',#7831);
#7833=FILL_AREA_STYLE('',(#7832));
#7834=SURFACE_STYLE_FILL_AREA(#7833);
#7835=SURFACE_SIDE_STYLE('',(#7834));
#7836=SURFACE_STYLE_USAGE(.BOTH.,#7835);
#7837=PRESENTATION_STYLE_ASSIGNMENT((#7836));
ENDSEC;
END-ISO-10303-21;
